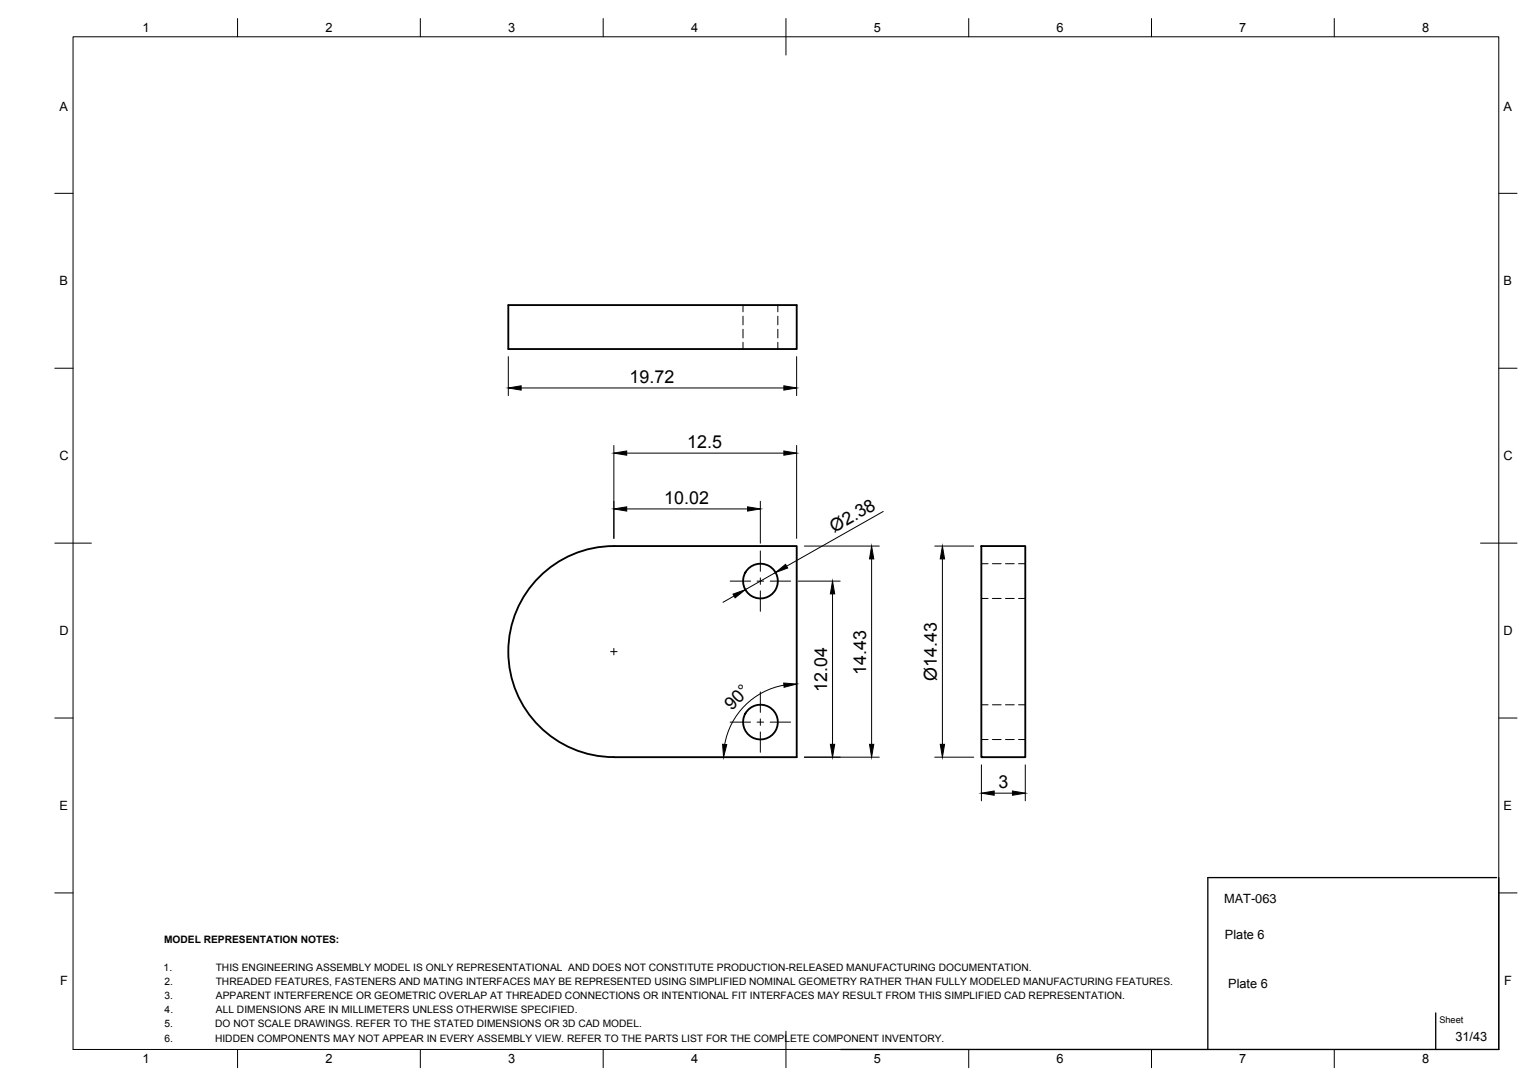
ISO-10303-21;
HEADER;
/* Generated by software containing ST-Developer
 * from STEP Tools, Inc. (www.steptools.com) 
 */

FILE_DESCRIPTION(
/* description */ (''),
/* implementation_level */ '2;1');

FILE_NAME(
/* name */ 'Plate 6.step',
/* time_stamp */ '2026-10-24T09:43:01-07:00',
/* author */ (''),
/* organization */ (''),
/* preprocessor_version */ 'ST-DEVELOPER v20.2',
/* originating_system */ 'Autodesk Translation Framework v15.15.0.0',
/* authorisation */ '');

FILE_SCHEMA (('AUTOMOTIVE_DESIGN { 1 0 10303 214 3 1 1 }'));
ENDSEC;

DATA;
#10=MECHANICAL_DESIGN_GEOMETRIC_PRESENTATION_REPRESENTATION('',(#296),#11112);
#230=SHAPE_REPRESENTATION_RELATIONSHIP('SRR','None',#11255,#263);
#263=ADVANCED_BREP_SHAPE_REPRESENTATION('',(#329),#11100);
#296=STYLED_ITEM('',(#11426),#329);
#329=MANIFOLD_SOLID_BREP('Plate 6',#6033);
#475=FACE_BOUND('',#1491,.T.);
#476=FACE_BOUND('',#1492,.T.);
#477=FACE_BOUND('',#1499,.T.);
#478=FACE_BOUND('',#1500,.T.);
#643=PLANE('',#7126);
#644=PLANE('',#7131);
#645=PLANE('',#7134);
#646=PLANE('',#7135);
#647=PLANE('',#7136);
#989=FACE_OUTER_BOUND('',#1489,.T.);
#990=FACE_OUTER_BOUND('',#1490,.T.);
#991=FACE_OUTER_BOUND('',#1493,.T.);
#992=FACE_OUTER_BOUND('',#1494,.T.);
#993=FACE_OUTER_BOUND('',#1495,.T.);
#994=FACE_OUTER_BOUND('',#1496,.T.);
#995=FACE_OUTER_BOUND('',#1497,.T.);
#996=FACE_OUTER_BOUND('',#1498,.T.);
#1489=EDGE_LOOP('',(#5329,#5330,#5331,#5332));
#1490=EDGE_LOOP('',(#5333,#5334,#5335,#5336));
#1491=EDGE_LOOP('',(#5337));
#1492=EDGE_LOOP('',(#5338));
#1493=EDGE_LOOP('',(#5339,#5340,#5341,#5342));
#1494=EDGE_LOOP('',(#5343,#5344,#5345,#5346));
#1495=EDGE_LOOP('',(#5347,#5348,#5349,#5350));
#1496=EDGE_LOOP('',(#5351,#5352,#5353,#5354));
#1497=EDGE_LOOP('',(#5355,#5356,#5357,#5358));
#1498=EDGE_LOOP('',(#5359,#5360,#5361,#5362));
#1499=EDGE_LOOP('',(#5363));
#1500=EDGE_LOOP('',(#5364));
#1880=LINE('',#10807,#2239);
#1881=LINE('',#10812,#2240);
#1882=LINE('',#10814,#2241);
#1883=LINE('',#10817,#2242);
#1884=LINE('',#10822,#2243);
#1885=LINE('',#10826,#2244);
#1886=LINE('',#10828,#2245);
#1887=LINE('',#10829,#2246);
#1888=LINE('',#10832,#2247);
#1889=LINE('',#10836,#2248);
#1890=LINE('',#10837,#2249);
#1891=LINE('',#10839,#2250);
#2239=VECTOR('',#9018,0.00118970000000007);
#2240=VECTOR('',#9023,0.01);
#2241=VECTOR('',#9024,0.01);
#2242=VECTOR('',#9027,0.01);
#2243=VECTOR('',#9032,0.00118970100000004);
#2244=VECTOR('',#9037,0.01);
#2245=VECTOR('',#9038,0.01);
#2246=VECTOR('',#9039,0.01);
#2247=VECTOR('',#9042,0.01);
#2248=VECTOR('',#9047,0.01);
#2249=VECTOR('',#9048,0.01);
#2250=VECTOR('',#9051,0.01);
#2642=CIRCLE('',#7124,0.00118970000000007);
#2643=CIRCLE('',#7125,0.00118970000000007);
#2644=CIRCLE('',#7127,0.007216878);
#2645=CIRCLE('',#7128,0.00118970100000004);
#2646=CIRCLE('',#7130,0.00118970100000004);
#2647=CIRCLE('',#7133,0.007216878);
#3122=VERTEX_POINT('',#10804);
#3123=VERTEX_POINT('',#10806);
#3124=VERTEX_POINT('',#10810);
#3125=VERTEX_POINT('',#10811);
#3126=VERTEX_POINT('',#10813);
#3127=VERTEX_POINT('',#10815);
#3128=VERTEX_POINT('',#10818);
#3129=VERTEX_POINT('',#10821);
#3130=VERTEX_POINT('',#10825);
#3131=VERTEX_POINT('',#10827);
#3132=VERTEX_POINT('',#10831);
#3133=VERTEX_POINT('',#10835);
#3868=EDGE_CURVE('',#3122,#3122,#2642,.T.);
#3869=EDGE_CURVE('',#3122,#3123,#1880,.T.);
#3870=EDGE_CURVE('',#3123,#3123,#2643,.F.);
#3871=EDGE_CURVE('',#3124,#3125,#1881,.T.);
#3872=EDGE_CURVE('',#3125,#3126,#1882,.T.);
#3873=EDGE_CURVE('',#3126,#3127,#2644,.F.);
#3874=EDGE_CURVE('',#3127,#3124,#1883,.T.);
#3875=EDGE_CURVE('',#3128,#3128,#2645,.T.);
#3876=EDGE_CURVE('',#3128,#3129,#1884,.T.);
#3877=EDGE_CURVE('',#3129,#3129,#2646,.F.);
#3878=EDGE_CURVE('',#3130,#3127,#1885,.T.);
#3879=EDGE_CURVE('',#3131,#3130,#1886,.T.);
#3880=EDGE_CURVE('',#3124,#3131,#1887,.T.);
#3881=EDGE_CURVE('',#3126,#3132,#1888,.F.);
#3882=EDGE_CURVE('',#3132,#3130,#2647,.F.);
#3883=EDGE_CURVE('',#3133,#3125,#1889,.T.);
#3884=EDGE_CURVE('',#3132,#3133,#1890,.T.);
#3885=EDGE_CURVE('',#3133,#3131,#1891,.T.);
#5329=ORIENTED_EDGE('',*,*,#3868,.F.);
#5330=ORIENTED_EDGE('',*,*,#3869,.T.);
#5331=ORIENTED_EDGE('',*,*,#3870,.F.);
#5332=ORIENTED_EDGE('',*,*,#3869,.F.);
#5333=ORIENTED_EDGE('',*,*,#3871,.T.);
#5334=ORIENTED_EDGE('',*,*,#3872,.T.);
#5335=ORIENTED_EDGE('',*,*,#3873,.T.);
#5336=ORIENTED_EDGE('',*,*,#3874,.T.);
#5337=ORIENTED_EDGE('',*,*,#3875,.T.);
#5338=ORIENTED_EDGE('',*,*,#3868,.T.);
#5339=ORIENTED_EDGE('',*,*,#3875,.F.);
#5340=ORIENTED_EDGE('',*,*,#3876,.T.);
#5341=ORIENTED_EDGE('',*,*,#3877,.F.);
#5342=ORIENTED_EDGE('',*,*,#3876,.F.);
#5343=ORIENTED_EDGE('',*,*,#3878,.F.);
#5344=ORIENTED_EDGE('',*,*,#3879,.F.);
#5345=ORIENTED_EDGE('',*,*,#3880,.F.);
#5346=ORIENTED_EDGE('',*,*,#3874,.F.);
#5347=ORIENTED_EDGE('',*,*,#3881,.T.);
#5348=ORIENTED_EDGE('',*,*,#3882,.T.);
#5349=ORIENTED_EDGE('',*,*,#3878,.T.);
#5350=ORIENTED_EDGE('',*,*,#3873,.F.);
#5351=ORIENTED_EDGE('',*,*,#3883,.F.);
#5352=ORIENTED_EDGE('',*,*,#3884,.F.);
#5353=ORIENTED_EDGE('',*,*,#3881,.F.);
#5354=ORIENTED_EDGE('',*,*,#3872,.F.);
#5355=ORIENTED_EDGE('',*,*,#3880,.T.);
#5356=ORIENTED_EDGE('',*,*,#3885,.F.);
#5357=ORIENTED_EDGE('',*,*,#3883,.T.);
#5358=ORIENTED_EDGE('',*,*,#3871,.F.);
#5359=ORIENTED_EDGE('',*,*,#3884,.T.);
#5360=ORIENTED_EDGE('',*,*,#3885,.T.);
#5361=ORIENTED_EDGE('',*,*,#3879,.T.);
#5362=ORIENTED_EDGE('',*,*,#3882,.F.);
#5363=ORIENTED_EDGE('',*,*,#3877,.T.);
#5364=ORIENTED_EDGE('',*,*,#3870,.T.);
#5620=CYLINDRICAL_SURFACE('',#7123,0.00118970000000007);
#5621=CYLINDRICAL_SURFACE('',#7129,0.00118970100000004);
#5622=CYLINDRICAL_SURFACE('',#7132,0.007216878);
#5962=ADVANCED_FACE('',(#989),#5620,.F.);
#5963=ADVANCED_FACE('',(#990,#475,#476),#643,.T.);
#5964=ADVANCED_FACE('',(#991),#5621,.F.);
#5965=ADVANCED_FACE('',(#992),#644,.F.);
#5966=ADVANCED_FACE('',(#993),#5622,.T.);
#5967=ADVANCED_FACE('',(#994),#645,.F.);
#5968=ADVANCED_FACE('',(#995),#646,.F.);
#5969=ADVANCED_FACE('',(#996,#477,#478),#647,.F.);
#6033=CLOSED_SHELL('',(#5962,#5963,#5964,#5965,#5966,#5967,#5968,#5969));
#7122=AXIS2_PLACEMENT_3D('',#10802,#9012,#9013);
#7123=AXIS2_PLACEMENT_3D('',#10803,#9014,#9015);
#7124=AXIS2_PLACEMENT_3D('',#10805,#9016,#9017);
#7125=AXIS2_PLACEMENT_3D('',#10808,#9019,#9020);
#7126=AXIS2_PLACEMENT_3D('',#10809,#9021,#9022);
#7127=AXIS2_PLACEMENT_3D('',#10816,#9025,#9026);
#7128=AXIS2_PLACEMENT_3D('',#10819,#9028,#9029);
#7129=AXIS2_PLACEMENT_3D('',#10820,#9030,#9031);
#7130=AXIS2_PLACEMENT_3D('',#10823,#9033,#9034);
#7131=AXIS2_PLACEMENT_3D('',#10824,#9035,#9036);
#7132=AXIS2_PLACEMENT_3D('',#10830,#9040,#9041);
#7133=AXIS2_PLACEMENT_3D('',#10833,#9043,#9044);
#7134=AXIS2_PLACEMENT_3D('',#10834,#9045,#9046);
#7135=AXIS2_PLACEMENT_3D('',#10838,#9049,#9050);
#7136=AXIS2_PLACEMENT_3D('',#10840,#9052,#9053);
#9012=DIRECTION('axis',(0.,0.,1.));
#9013=DIRECTION('refdir',(1.,0.,0.));
#9014=DIRECTION('center_axis',(-1.,0.,0.));
#9015=DIRECTION('ref_axis',(0.,0.,1.));
#9016=DIRECTION('center_axis',(-1.,0.,0.));
#9017=DIRECTION('ref_axis',(0.,0.,1.));
#9018=DIRECTION('',(-1.,0.,0.));
#9019=DIRECTION('center_axis',(-1.,0.,0.));
#9020=DIRECTION('ref_axis',(0.,0.,1.));
#9021=DIRECTION('center_axis',(1.,-4.4804899918026E-16,8.23217897544922E-17));
#9022=DIRECTION('ref_axis',(4.4804899918026E-16,1.,2.26725874505889E-48));
#9023=DIRECTION('',(0.,-0.49999998104077,0.866025414730555));
#9024=DIRECTION('',(5.68434220074081E-15,-0.866025412838334,-0.499999984318193));
#9025=DIRECTION('center_axis',(-1.,0.,0.));
#9026=DIRECTION('ref_axis',(0.,0.,1.));
#9027=DIRECTION('',(0.,0.866025392838327,0.500000018959221));
#9028=DIRECTION('center_axis',(-1.,0.,0.));
#9029=DIRECTION('ref_axis',(0.,0.,1.));
#9030=DIRECTION('center_axis',(-1.,0.,0.));
#9031=DIRECTION('ref_axis',(0.,0.,1.));
#9032=DIRECTION('',(-1.,0.,0.));
#9033=DIRECTION('center_axis',(-1.,0.,0.));
#9034=DIRECTION('ref_axis',(0.,0.,1.));
#9035=DIRECTION('center_axis',(-3.99107463157378E-15,-0.500000018959218,
0.866025392838329));
#9036=DIRECTION('ref_axis',(7.48434538625964E-32,-0.866025392838329,-0.500000018959218));
#9037=DIRECTION('',(1.,0.,0.));
#9038=DIRECTION('',(0.,-0.866025392838343,-0.500000018959194));
#9039=DIRECTION('',(-1.,0.,0.));
#9040=DIRECTION('center_axis',(-1.,0.,0.));
#9041=DIRECTION('ref_axis',(0.,-0.866025406570393,-0.499999995174586));
#9042=DIRECTION('',(1.,0.,0.));
#9043=DIRECTION('center_axis',(-1.,0.,0.));
#9044=DIRECTION('ref_axis',(0.,0.,1.));
#9045=DIRECTION('center_axis',(1.04209967862532E-14,0.499999984318195,-0.866025412838333));
#9046=DIRECTION('ref_axis',(4.87803011688087E-32,0.866025412838333,0.499999984318195));
#9047=DIRECTION('',(1.,0.,0.));
#9048=DIRECTION('',(0.,0.866025412838317,0.499999984318223));
#9049=DIRECTION('center_axis',(6.43478340347328E-15,-0.866025414730554,
-0.499999981040772));
#9050=DIRECTION('ref_axis',(6.55419316660567E-32,0.499999981040772,-0.866025414730554));
#9051=DIRECTION('',(0.,0.499999981040781,-0.866025414730549));
#9052=DIRECTION('center_axis',(1.,1.49593502589698E-15,6.8668419608312E-16));
#9053=DIRECTION('ref_axis',(-1.49593502589698E-15,1.,8.50544090484151E-47));
#10802=CARTESIAN_POINT('',(0.,0.,0.));
#10803=CARTESIAN_POINT('Origin',(-0.477,-0.542782557,0.975695518));
#10804=CARTESIAN_POINT('',(-0.477,-0.542782557,0.974505818));
#10805=CARTESIAN_POINT('Origin',(-0.477,-0.542782557,0.975695518));
#10806=CARTESIAN_POINT('',(-0.48,-0.542782557,0.974505818));
#10807=CARTESIAN_POINT('',(-0.477,-0.542782557,0.974505818));
#10808=CARTESIAN_POINT('Origin',(-0.48,-0.542782557,0.975695518));
#10809=CARTESIAN_POINT('Origin',(-0.477,-0.545454380845135,0.969136388159038));
#10810=CARTESIAN_POINT('',(-0.477,-0.534613544999688,0.966510345999423));
#10811=CARTESIAN_POINT('',(-0.477,-0.541830423000466,0.979010345999528));
#10812=CARTESIAN_POINT('',(-0.477,-0.534613544872232,0.9665103457787));
#10813=CARTESIAN_POINT('',(-0.477000000014632,-0.552655740191489,0.972760346019922));
#10814=CARTESIAN_POINT('',(-0.477,-0.541830423323753,0.979010345813081));
#10815=CARTESIAN_POINT('',(-0.477,-0.545438862110786,0.960260346041367));
#10816=CARTESIAN_POINT('Origin',(-0.477,-0.549047301,0.966510346));
#10817=CARTESIAN_POINT('',(-0.477,-0.545438862219975,0.960260345872998));
#10818=CARTESIAN_POINT('',(-0.477,-0.537960337,0.966153487));
#10819=CARTESIAN_POINT('Origin',(-0.477,-0.537960337,0.967343188));
#10820=CARTESIAN_POINT('Origin',(-0.477,-0.537960337,0.967343188));
#10821=CARTESIAN_POINT('',(-0.48,-0.537960337,0.966153487));
#10822=CARTESIAN_POINT('',(-0.477,-0.537960337,0.966153487));
#10823=CARTESIAN_POINT('Origin',(-0.48,-0.537960337,0.967343188));
#10824=CARTESIAN_POINT('Origin',(-0.4785,-0.5400262035,0.963385346000001));
#10825=CARTESIAN_POINT('',(-0.48,-0.545438861975815,0.960260346119293));
#10826=CARTESIAN_POINT('',(-0.479999999999999,-0.545438862,0.960260346000001));
#10827=CARTESIAN_POINT('',(-0.479999999999999,-0.53461354500041,0.966510345999764));
#10828=CARTESIAN_POINT('',(-0.479999999999999,-0.534613545008309,0.966510345995204));
#10829=CARTESIAN_POINT('',(-0.476999999999999,-0.534613545,0.966510346000001));
#10830=CARTESIAN_POINT('Origin',(-0.477,-0.549047301,0.966510346));
#10831=CARTESIAN_POINT('',(-0.48,-0.552655740263515,0.972760345829652));
#10832=CARTESIAN_POINT('',(-0.47999999975,-0.552655739997383,0.972760345685524));
#10833=CARTESIAN_POINT('Origin',(-0.48,-0.549047301,0.966510346));
#10834=CARTESIAN_POINT('Origin',(-0.4785,-0.547243082,0.975885346));
#10835=CARTESIAN_POINT('',(-0.48,-0.541830423,0.979010346));
#10836=CARTESIAN_POINT('',(-0.479999999999999,-0.541830423,0.979010346));
#10837=CARTESIAN_POINT('',(-0.479999999999999,-0.552655740692886,0.972760346177312));
#10838=CARTESIAN_POINT('Origin',(-0.4785,-0.538221983999999,0.972760345999999));
#10839=CARTESIAN_POINT('',(-0.479999999999999,-0.541830422999999,0.979010346));
#10840=CARTESIAN_POINT('Origin',(-0.48,-0.545454380845135,0.969136388159038));
#11061=UNCERTAINTY_MEASURE_WITH_UNIT(LENGTH_MEASURE(1.E-5),#11113,
'DISTANCE_ACCURACY_VALUE',
'Maximum model space distance between geometric entities at asserted c
onnectivities');
#11073=UNCERTAINTY_MEASURE_WITH_UNIT(LENGTH_MEASURE(1.E-5),#11113,
'DISTANCE_ACCURACY_VALUE',
'Maximum model space distance between geometric entities at asserted c
onnectivities');
#11100=(
GEOMETRIC_REPRESENTATION_CONTEXT(3)
GLOBAL_UNCERTAINTY_ASSIGNED_CONTEXT((#11061))
GLOBAL_UNIT_ASSIGNED_CONTEXT((#11113,#11114,#11115))
REPRESENTATION_CONTEXT('','3D')
);
#11112=(
GEOMETRIC_REPRESENTATION_CONTEXT(3)
GLOBAL_UNCERTAINTY_ASSIGNED_CONTEXT((#11073))
GLOBAL_UNIT_ASSIGNED_CONTEXT((#11113,#11114,#11115))
REPRESENTATION_CONTEXT('','3D')
);
#11113=(
LENGTH_UNIT()
NAMED_UNIT(*)
SI_UNIT($,.METRE.)
);
#11114=(
NAMED_UNIT(*)
PLANE_ANGLE_UNIT()
SI_UNIT($,.RADIAN.)
);
#11115=(
NAMED_UNIT(*)
SI_UNIT($,.STERADIAN.)
SOLID_ANGLE_UNIT()
);
#11142=SHAPE_DEFINITION_REPRESENTATION(#11187,#11255);
#11187=PRODUCT_DEFINITION_SHAPE('',$,#11294);
#11255=SHAPE_REPRESENTATION('',(#7122),#11100);
#11267=PRODUCT_DEFINITION_CONTEXT('part definition',#11383,'design');
#11294=PRODUCT_DEFINITION('Plate 6','Plate 6',#11332,#11267);
#11332=PRODUCT_DEFINITION_FORMATION('',$,#11411);
#11383=APPLICATION_CONTEXT(
'Core Data for Automotive Mechanical Design Process');
#11384=PRODUCT_CONTEXT('part definition',#11383,'mechanical');
#11411=PRODUCT('Plate 6','Plate 6','all_plates__ DE     1187',(#11384));
#11426=PRESENTATION_STYLE_ASSIGNMENT((#11430));
#11430=SURFACE_STYLE_USAGE(.BOTH.,#11434);
#11434=SURFACE_SIDE_STYLE('',(#11438));
#11438=SURFACE_STYLE_FILL_AREA(#11442);
#11442=FILL_AREA_STYLE('Opaque(202,209,238)',(#11446));
#11446=FILL_AREA_STYLE_COLOUR('Opaque(202,209,238)',#11450);
#11450=COLOUR_RGB('Opaque(202,209,238)',0.792156862745098,0.819607843137255,
0.933333333333333);
ENDSEC;
END-ISO-10303-21;
